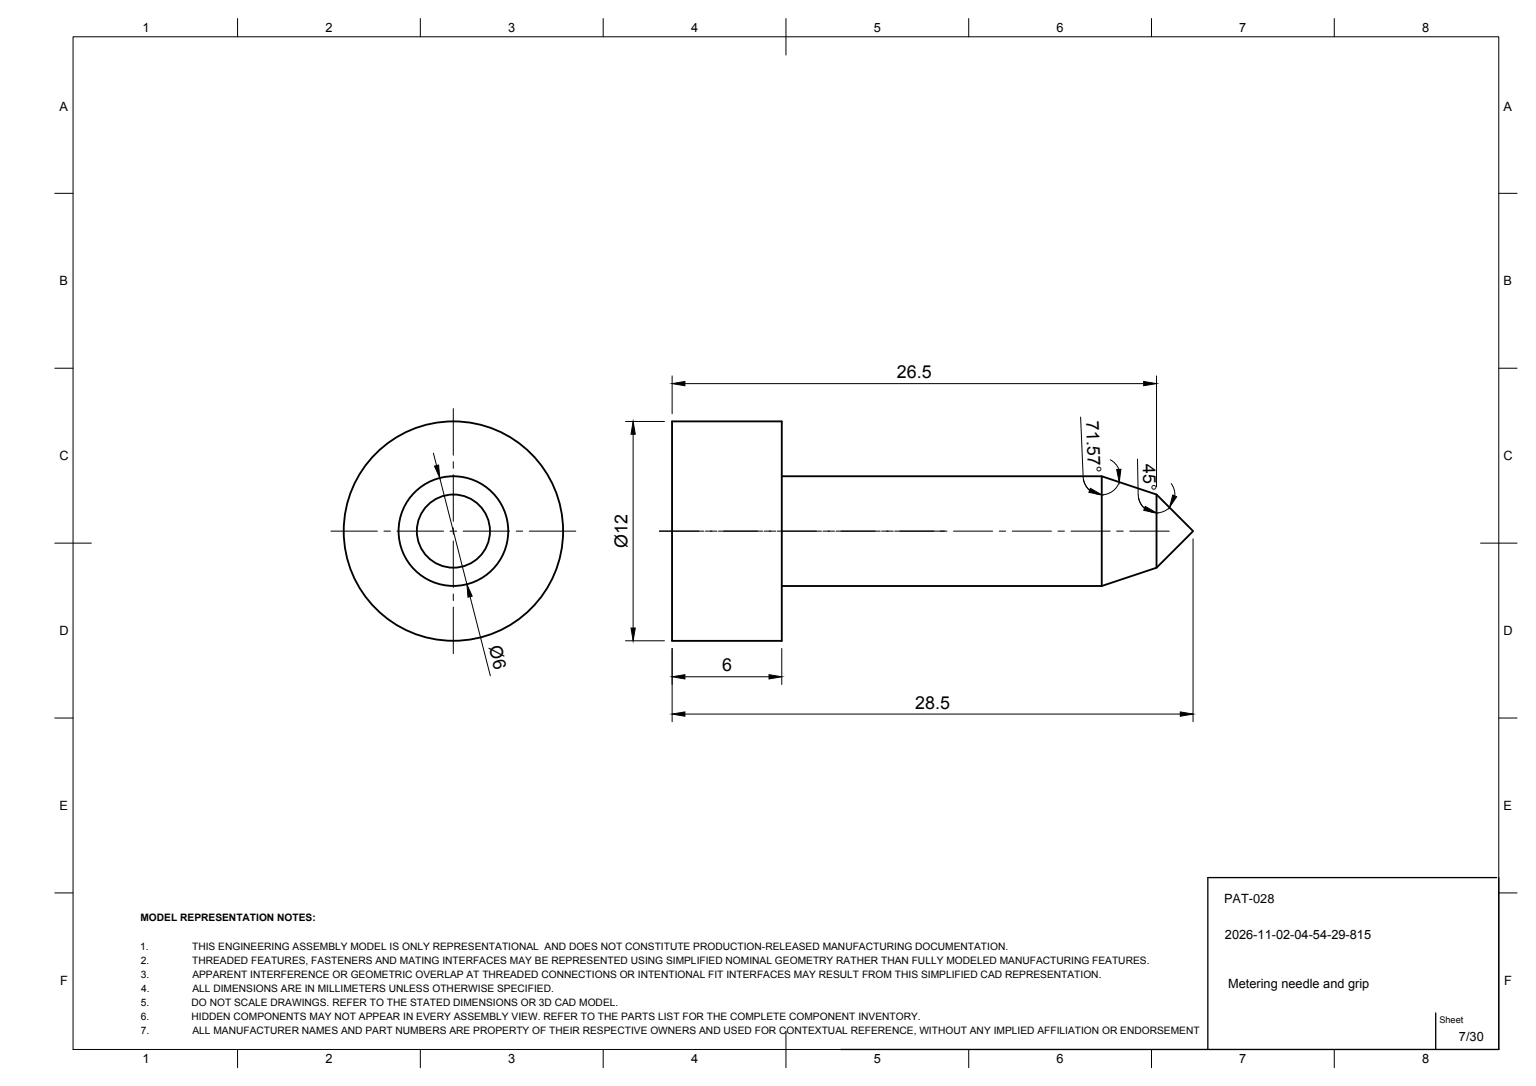
ISO-10303-21;
HEADER;
/* Generated by software containing ST-Developer
 * from STEP Tools, Inc. (www.steptools.com) 
 */

FILE_DESCRIPTION(
/* description */ ('Cylinder foot and clevis mount kit'),
/* implementation_level */ '2;1');

FILE_NAME(
/* name */ 'Metering needle and grip.step',
/* time_stamp */ '2026-10-27T20:10:43-07:00',
/* author */ (''),
/* organization */ (''),
/* preprocessor_version */ 'ST-DEVELOPER v20.2',
/* originating_system */ 'Autodesk Translation Framework v15.17.0.0',
/* authorisation */ '');

FILE_SCHEMA (('AUTOMOTIVE_DESIGN { 1 0 10303 214 3 1 1 }'));
ENDSEC;

DATA;
#10=MECHANICAL_DESIGN_GEOMETRIC_PRESENTATION_REPRESENTATION('',(#340),#9102);
#263=CONICAL_SURFACE('',#5380,0.1,0.78539816339745);
#264=CONICAL_SURFACE('',#5382,0.25,0.321750554396641);
#284=SHAPE_REPRESENTATION_RELATIONSHIP('SRR','None',#9231,#312);
#312=ADVANCED_BREP_SHAPE_REPRESENTATION('',(#368),#9074);
#340=STYLED_ITEM('',(#9467),#368);
#368=MANIFOLD_SOLID_BREP('Body1',#4926);
#416=FACE_BOUND('',#1090,.T.);
#548=PLANE('',#5386);
#549=PLANE('',#5390);
#756=FACE_OUTER_BOUND('',#1086,.T.);
#757=FACE_OUTER_BOUND('',#1087,.T.);
#758=FACE_OUTER_BOUND('',#1088,.T.);
#759=FACE_OUTER_BOUND('',#1089,.T.);
#760=FACE_OUTER_BOUND('',#1091,.T.);
#761=FACE_OUTER_BOUND('',#1092,.T.);
#1086=EDGE_LOOP('',(#3573,#3574,#3575));
#1087=EDGE_LOOP('',(#3576,#3577,#3578,#3579));
#1088=EDGE_LOOP('',(#3580,#3581,#3582,#3583));
#1089=EDGE_LOOP('',(#3584));
#1090=EDGE_LOOP('',(#3585));
#1091=EDGE_LOOP('',(#3586,#3587,#3588,#3589));
#1092=EDGE_LOOP('',(#3590));
#1488=LINE('',#7775,#1837);
#1489=LINE('',#7779,#1838);
#1490=LINE('',#7783,#1839);
#1491=LINE('',#7790,#1840);
#1837=VECTOR('',#6207,0.1);
#1838=VECTOR('',#6212,0.25);
#1839=VECTOR('',#6217,0.3);
#1840=VECTOR('',#6226,0.6);
#2152=CIRCLE('',#5381,0.2);
#2153=CIRCLE('',#5383,0.3);
#2154=CIRCLE('',#5385,0.3);
#2155=CIRCLE('',#5387,0.6);
#2156=CIRCLE('',#5389,0.6);
#2408=VERTEX_POINT('',#7772);
#2409=VERTEX_POINT('',#7774);
#2410=VERTEX_POINT('',#7777);
#2411=VERTEX_POINT('',#7781);
#2412=VERTEX_POINT('',#7785);
#2413=VERTEX_POINT('',#7788);
#2841=EDGE_CURVE('',#2408,#2408,#2152,.T.);
#2842=EDGE_CURVE('',#2408,#2409,#1488,.T.);
#2843=EDGE_CURVE('',#2410,#2410,#2153,.T.);
#2844=EDGE_CURVE('',#2410,#2408,#1489,.T.);
#2845=EDGE_CURVE('',#2411,#2411,#2154,.T.);
#2846=EDGE_CURVE('',#2411,#2410,#1490,.T.);
#2847=EDGE_CURVE('',#2412,#2412,#2155,.T.);
#2848=EDGE_CURVE('',#2413,#2413,#2156,.T.);
#2849=EDGE_CURVE('',#2413,#2412,#1491,.T.);
#3573=ORIENTED_EDGE('',*,*,#2841,.F.);
#3574=ORIENTED_EDGE('',*,*,#2842,.T.);
#3575=ORIENTED_EDGE('',*,*,#2842,.F.);
#3576=ORIENTED_EDGE('',*,*,#2843,.F.);
#3577=ORIENTED_EDGE('',*,*,#2844,.T.);
#3578=ORIENTED_EDGE('',*,*,#2841,.T.);
#3579=ORIENTED_EDGE('',*,*,#2844,.F.);
#3580=ORIENTED_EDGE('',*,*,#2845,.F.);
#3581=ORIENTED_EDGE('',*,*,#2846,.T.);
#3582=ORIENTED_EDGE('',*,*,#2843,.T.);
#3583=ORIENTED_EDGE('',*,*,#2846,.F.);
#3584=ORIENTED_EDGE('',*,*,#2847,.F.);
#3585=ORIENTED_EDGE('',*,*,#2845,.T.);
#3586=ORIENTED_EDGE('',*,*,#2848,.F.);
#3587=ORIENTED_EDGE('',*,*,#2849,.T.);
#3588=ORIENTED_EDGE('',*,*,#2847,.T.);
#3589=ORIENTED_EDGE('',*,*,#2849,.F.);
#3590=ORIENTED_EDGE('',*,*,#2848,.T.);
#4543=CYLINDRICAL_SURFACE('',#5384,0.3);
#4544=CYLINDRICAL_SURFACE('',#5388,0.6);
#4679=ADVANCED_FACE('',(#756),#263,.T.);
#4680=ADVANCED_FACE('',(#757),#264,.T.);
#4681=ADVANCED_FACE('',(#758),#4543,.T.);
#4682=ADVANCED_FACE('',(#759,#416),#548,.T.);
#4683=ADVANCED_FACE('',(#760),#4544,.T.);
#4684=ADVANCED_FACE('',(#761),#549,.T.);
#4926=CLOSED_SHELL('',(#4679,#4680,#4681,#4682,#4683,#4684));
#5379=AXIS2_PLACEMENT_3D('',#7770,#6201,#6202);
#5380=AXIS2_PLACEMENT_3D('',#7771,#6203,#6204);
#5381=AXIS2_PLACEMENT_3D('',#7773,#6205,#6206);
#5382=AXIS2_PLACEMENT_3D('',#7776,#6208,#6209);
#5383=AXIS2_PLACEMENT_3D('',#7778,#6210,#6211);
#5384=AXIS2_PLACEMENT_3D('',#7780,#6213,#6214);
#5385=AXIS2_PLACEMENT_3D('',#7782,#6215,#6216);
#5386=AXIS2_PLACEMENT_3D('',#7784,#6218,#6219);
#5387=AXIS2_PLACEMENT_3D('',#7786,#6220,#6221);
#5388=AXIS2_PLACEMENT_3D('',#7787,#6222,#6223);
#5389=AXIS2_PLACEMENT_3D('',#7789,#6224,#6225);
#5390=AXIS2_PLACEMENT_3D('',#7791,#6227,#6228);
#6201=DIRECTION('axis',(0.,0.,1.));
#6202=DIRECTION('refdir',(1.,0.,0.));
#6203=DIRECTION('center_axis',(0.,0.,1.));
#6204=DIRECTION('ref_axis',(1.,0.,0.));
#6205=DIRECTION('center_axis',(0.,0.,1.));
#6206=DIRECTION('ref_axis',(1.,0.,0.));
#6207=DIRECTION('',(0.707106781186549,8.65956056235495E-17,-0.707106781186546));
#6208=DIRECTION('center_axis',(0.,0.,1.));
#6209=DIRECTION('ref_axis',(1.,0.,0.));
#6210=DIRECTION('center_axis',(0.,0.,1.));
#6211=DIRECTION('ref_axis',(1.,0.,0.));
#6212=DIRECTION('',(0.316227766016837,3.87267321454038E-17,-0.948683298050514));
#6213=DIRECTION('center_axis',(0.,0.,1.));
#6214=DIRECTION('ref_axis',(1.,0.,0.));
#6215=DIRECTION('center_axis',(0.,0.,1.));
#6216=DIRECTION('ref_axis',(1.,0.,0.));
#6217=DIRECTION('',(0.,0.,-1.));
#6218=DIRECTION('center_axis',(0.,0.,-1.));
#6219=DIRECTION('ref_axis',(-1.,0.,0.));
#6220=DIRECTION('center_axis',(0.,0.,1.));
#6221=DIRECTION('ref_axis',(1.,0.,0.));
#6222=DIRECTION('center_axis',(0.,0.,1.));
#6223=DIRECTION('ref_axis',(1.,0.,0.));
#6224=DIRECTION('center_axis',(0.,0.,1.));
#6225=DIRECTION('ref_axis',(1.,0.,0.));
#6226=DIRECTION('',(0.,0.,-1.));
#6227=DIRECTION('center_axis',(0.,0.,1.));
#6228=DIRECTION('ref_axis',(1.,0.,0.));
#7770=CARTESIAN_POINT('',(0.,0.,0.));
#7771=CARTESIAN_POINT('Origin',(0.,0.8,8.15));
#7772=CARTESIAN_POINT('',(-0.2,0.8,8.25));
#7773=CARTESIAN_POINT('Origin',(0.,0.8,8.25));
#7774=CARTESIAN_POINT('',(0.,0.8,8.05));
#7775=CARTESIAN_POINT('',(-0.1,0.8,8.15));
#7776=CARTESIAN_POINT('Origin',(0.,0.8,8.4));
#7777=CARTESIAN_POINT('',(-0.3,0.8,8.55));
#7778=CARTESIAN_POINT('Origin',(0.,0.8,8.55));
#7779=CARTESIAN_POINT('',(-0.25,0.8,8.4));
#7780=CARTESIAN_POINT('Origin',(0.,0.8,9.425));
#7781=CARTESIAN_POINT('',(-0.3,0.8,10.3));
#7782=CARTESIAN_POINT('Origin',(0.,0.8,10.3));
#7783=CARTESIAN_POINT('',(-0.3,0.8,9.425));
#7784=CARTESIAN_POINT('Origin',(0.6,0.8,10.3));
#7785=CARTESIAN_POINT('',(-0.6,0.8,10.3));
#7786=CARTESIAN_POINT('Origin',(0.,0.8,10.3));
#7787=CARTESIAN_POINT('Origin',(0.,0.8,10.6));
#7788=CARTESIAN_POINT('',(-0.6,0.8,10.9));
#7789=CARTESIAN_POINT('Origin',(0.,0.8,10.9));
#7790=CARTESIAN_POINT('',(-0.6,0.8,10.6));
#7791=CARTESIAN_POINT('Origin',(0.,0.8,10.9));
#9041=UNCERTAINTY_MEASURE_WITH_UNIT(LENGTH_MEASURE(0.001),#9103,
'DISTANCE_ACCURACY_VALUE',
'Maximum model space distance between geometric entities at asserted c
onnectivities');
#9069=UNCERTAINTY_MEASURE_WITH_UNIT(LENGTH_MEASURE(0.001),#9103,
'DISTANCE_ACCURACY_VALUE',
'Maximum model space distance between geometric entities at asserted c
onnectivities');
#9074=(
GEOMETRIC_REPRESENTATION_CONTEXT(3)
GLOBAL_UNCERTAINTY_ASSIGNED_CONTEXT((#9041))
GLOBAL_UNIT_ASSIGNED_CONTEXT((#9103,#9105,#9106))
REPRESENTATION_CONTEXT('','3D')
);
#9102=(
GEOMETRIC_REPRESENTATION_CONTEXT(3)
GLOBAL_UNCERTAINTY_ASSIGNED_CONTEXT((#9069))
GLOBAL_UNIT_ASSIGNED_CONTEXT((#9103,#9105,#9106))
REPRESENTATION_CONTEXT('','3D')
);
#9103=(
LENGTH_UNIT()
NAMED_UNIT(*)
SI_UNIT(.CENTI.,.METRE.)
);
#9105=(
NAMED_UNIT(*)
PLANE_ANGLE_UNIT()
SI_UNIT($,.RADIAN.)
);
#9106=(
NAMED_UNIT(*)
SI_UNIT($,.STERADIAN.)
SOLID_ANGLE_UNIT()
);
#9111=SHAPE_DEFINITION_REPRESENTATION(#9143,#9231);
#9143=PRODUCT_DEFINITION_SHAPE('',$,#9264);
#9231=SHAPE_REPRESENTATION('',(#5379),#9074);
#9259=PRODUCT_DEFINITION_CONTEXT('part definition',#9357,'design');
#9264=PRODUCT_DEFINITION('Metering needle and grip',
'Metering needle and grip',#9296,#9259);
#9296=PRODUCT_DEFINITION_FORMATION('',$,#9363);
#9357=APPLICATION_CONTEXT(
'Core Data for Automotive Mechanical Design Process');
#9358=PRODUCT_CONTEXT('part definition',#9357,'mechanical');
#9363=PRODUCT('Metering needle and grip','Metering needle and grip',
'Metering needle and grip',(#9358));
#9461=COLOUR_RGB('Black',0.12,0.14,0.17);
#9462=FILL_AREA_STYLE_COLOUR('',#9461);
#9463=FILL_AREA_STYLE('',(#9462));
#9464=SURFACE_STYLE_FILL_AREA(#9463);
#9465=SURFACE_SIDE_STYLE('',(#9464));
#9466=SURFACE_STYLE_USAGE(.BOTH.,#9465);
#9467=PRESENTATION_STYLE_ASSIGNMENT((#9466));
ENDSEC;
END-ISO-10303-21;
